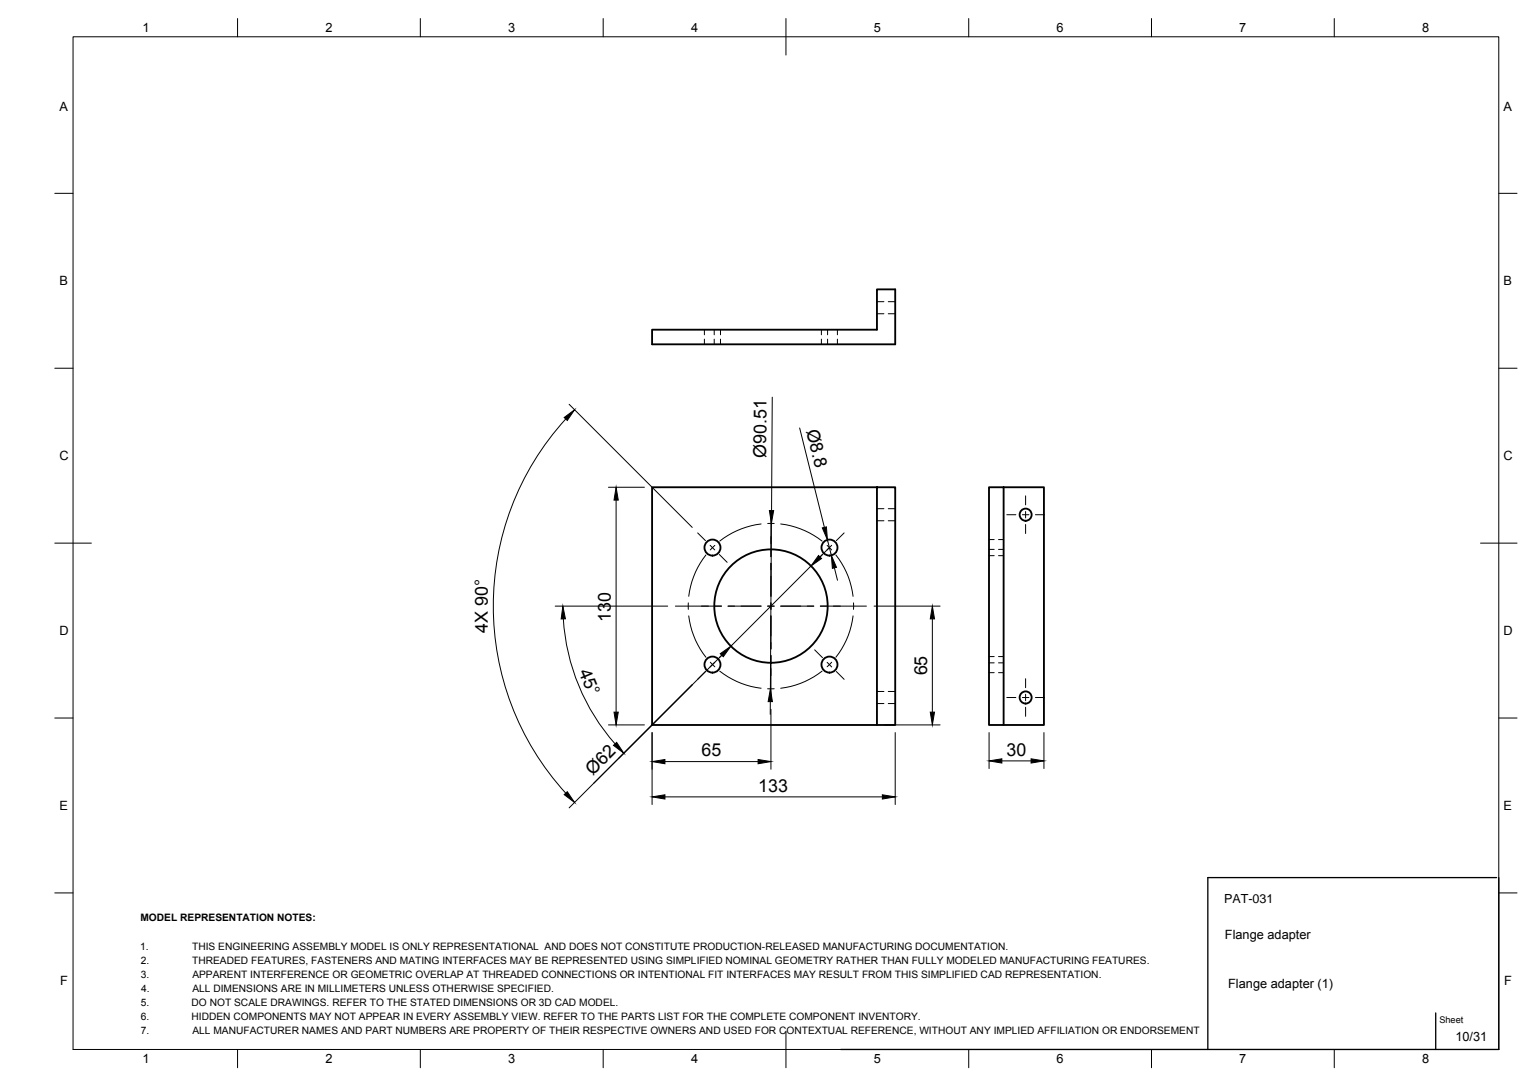
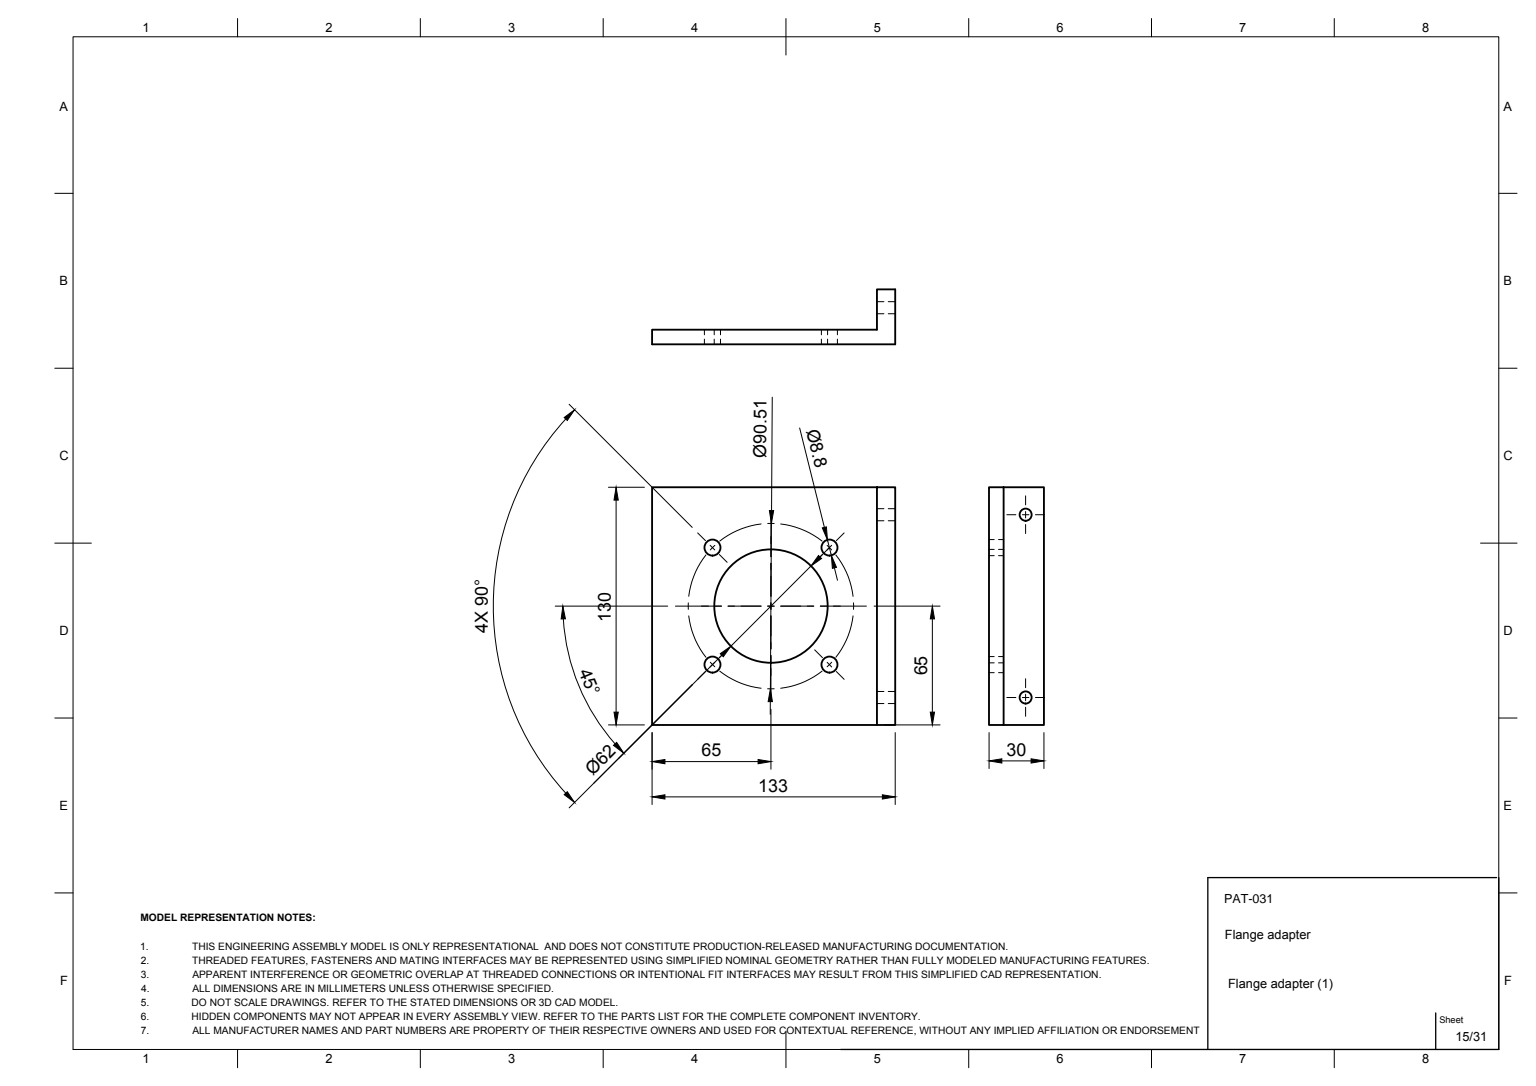
ISO-10303-21;
HEADER;
/* Generated by software containing ST-Developer
 * from STEP Tools, Inc. (www.steptools.com) 
 */

FILE_DESCRIPTION(
/* description */ ('Double-row support with tensioned shaft'),
/* implementation_level */ '2;1');

FILE_NAME(
/* name */ 'Flange adapter.step',
/* time_stamp */ '2026-10-27T10:50:35-07:00',
/* author */ (''),
/* organization */ (''),
/* preprocessor_version */ 'ST-DEVELOPER v20.2',
/* originating_system */ 'Autodesk Translation Framework v15.17.0.0',
/* authorisation */ '');

FILE_SCHEMA (('AUTOMOTIVE_DESIGN { 1 0 10303 214 3 1 1 }'));
ENDSEC;

DATA;
#10=MECHANICAL_DESIGN_GEOMETRIC_PRESENTATION_REPRESENTATION('',(#484),#11559);
#420=SHAPE_REPRESENTATION_RELATIONSHIP('SRR','None',#11728,#452);
#452=ADVANCED_BREP_SHAPE_REPRESENTATION('',(#517),#11530);
#484=STYLED_ITEM('',(#11953),#517);
#517=MANIFOLD_SOLID_BREP('Body1',#6329);
#566=FACE_BOUND('',#1335,.T.);
#567=FACE_BOUND('',#1336,.T.);
#568=FACE_BOUND('',#1339,.T.);
#569=FACE_BOUND('',#1340,.T.);
#570=FACE_BOUND('',#1341,.T.);
#571=FACE_BOUND('',#1342,.T.);
#572=FACE_BOUND('',#1343,.T.);
#573=FACE_BOUND('',#1347,.T.);
#574=FACE_BOUND('',#1348,.T.);
#575=FACE_BOUND('',#1349,.T.);
#576=FACE_BOUND('',#1350,.T.);
#577=FACE_BOUND('',#1351,.T.);
#578=FACE_BOUND('',#1354,.T.);
#579=FACE_BOUND('',#1355,.T.);
#709=PLANE('',#6808);
#710=PLANE('',#6809);
#711=PLANE('',#6810);
#712=PLANE('',#6811);
#713=PLANE('',#6812);
#714=PLANE('',#6813);
#715=PLANE('',#6814);
#716=PLANE('',#6815);
#959=FACE_OUTER_BOUND('',#1327,.T.);
#960=FACE_OUTER_BOUND('',#1328,.T.);
#961=FACE_OUTER_BOUND('',#1329,.T.);
#962=FACE_OUTER_BOUND('',#1330,.T.);
#963=FACE_OUTER_BOUND('',#1331,.T.);
#964=FACE_OUTER_BOUND('',#1332,.T.);
#965=FACE_OUTER_BOUND('',#1333,.T.);
#966=FACE_OUTER_BOUND('',#1334,.T.);
#967=FACE_OUTER_BOUND('',#1337,.T.);
#968=FACE_OUTER_BOUND('',#1338,.T.);
#969=FACE_OUTER_BOUND('',#1344,.T.);
#970=FACE_OUTER_BOUND('',#1345,.T.);
#971=FACE_OUTER_BOUND('',#1346,.T.);
#972=FACE_OUTER_BOUND('',#1352,.T.);
#973=FACE_OUTER_BOUND('',#1353,.T.);
#1327=EDGE_LOOP('',(#4522,#4523,#4524,#4525));
#1328=EDGE_LOOP('',(#4526,#4527,#4528,#4529));
#1329=EDGE_LOOP('',(#4530,#4531,#4532,#4533));
#1330=EDGE_LOOP('',(#4534,#4535,#4536,#4537));
#1331=EDGE_LOOP('',(#4538,#4539,#4540,#4541));
#1332=EDGE_LOOP('',(#4542,#4543,#4544,#4545));
#1333=EDGE_LOOP('',(#4546,#4547,#4548,#4549));
#1334=EDGE_LOOP('',(#4550,#4551,#4552,#4553));
#1335=EDGE_LOOP('',(#4554));
#1336=EDGE_LOOP('',(#4555));
#1337=EDGE_LOOP('',(#4556,#4557,#4558,#4559));
#1338=EDGE_LOOP('',(#4560,#4561,#4562,#4563));
#1339=EDGE_LOOP('',(#4564));
#1340=EDGE_LOOP('',(#4565));
#1341=EDGE_LOOP('',(#4566));
#1342=EDGE_LOOP('',(#4567));
#1343=EDGE_LOOP('',(#4568));
#1344=EDGE_LOOP('',(#4569,#4570,#4571,#4572,#4573,#4574));
#1345=EDGE_LOOP('',(#4575,#4576,#4577,#4578,#4579,#4580));
#1346=EDGE_LOOP('',(#4581,#4582,#4583,#4584));
#1347=EDGE_LOOP('',(#4585));
#1348=EDGE_LOOP('',(#4586));
#1349=EDGE_LOOP('',(#4587));
#1350=EDGE_LOOP('',(#4588));
#1351=EDGE_LOOP('',(#4589));
#1352=EDGE_LOOP('',(#4590,#4591,#4592,#4593));
#1353=EDGE_LOOP('',(#4594,#4595,#4596,#4597));
#1354=EDGE_LOOP('',(#4598));
#1355=EDGE_LOOP('',(#4599));
#1814=LINE('',#9448,#2361);
#1815=LINE('',#9454,#2362);
#1816=LINE('',#9460,#2363);
#1817=LINE('',#9466,#2364);
#1818=LINE('',#9472,#2365);
#1819=LINE('',#9478,#2366);
#1820=LINE('',#9484,#2367);
#1821=LINE('',#9489,#2368);
#1822=LINE('',#9491,#2369);
#1823=LINE('',#9493,#2370);
#1824=LINE('',#9494,#2371);
#1825=LINE('',#9497,#2372);
#1826=LINE('',#9499,#2373);
#1827=LINE('',#9500,#2374);
#1828=LINE('',#9504,#2375);
#1829=LINE('',#9506,#2376);
#1830=LINE('',#9508,#2377);
#1831=LINE('',#9509,#2378);
#1832=LINE('',#9512,#2379);
#1833=LINE('',#9513,#2380);
#1834=LINE('',#9514,#2381);
#1835=LINE('',#9517,#2382);
#1836=LINE('',#9518,#2383);
#1837=LINE('',#9519,#2384);
#1838=LINE('',#9521,#2385);
#2361=VECTOR('',#7595,0.33);
#2362=VECTOR('',#7602,0.33);
#2363=VECTOR('',#7609,0.44);
#2364=VECTOR('',#7616,0.44);
#2365=VECTOR('',#7623,0.44);
#2366=VECTOR('',#7630,0.44);
#2367=VECTOR('',#7637,3.1);
#2368=VECTOR('',#7642,1.);
#2369=VECTOR('',#7643,1.);
#2370=VECTOR('',#7644,1.);
#2371=VECTOR('',#7645,1.);
#2372=VECTOR('',#7648,1.);
#2373=VECTOR('',#7649,1.);
#2374=VECTOR('',#7650,1.);
#2375=VECTOR('',#7653,1.);
#2376=VECTOR('',#7654,1.);
#2377=VECTOR('',#7655,1.);
#2378=VECTOR('',#7656,1.);
#2379=VECTOR('',#7659,1.);
#2380=VECTOR('',#7660,1.);
#2381=VECTOR('',#7661,1.);
#2382=VECTOR('',#7664,1.);
#2383=VECTOR('',#7665,1.);
#2384=VECTOR('',#7666,1.);
#2385=VECTOR('',#7669,1.);
#2860=CIRCLE('',#6788,0.33);
#2861=CIRCLE('',#6789,0.33);
#2862=CIRCLE('',#6791,0.33);
#2863=CIRCLE('',#6792,0.33);
#2864=CIRCLE('',#6794,0.44);
#2865=CIRCLE('',#6795,0.44);
#2866=CIRCLE('',#6797,0.44);
#2867=CIRCLE('',#6798,0.44);
#2868=CIRCLE('',#6800,0.44);
#2869=CIRCLE('',#6801,0.44);
#2870=CIRCLE('',#6803,0.44);
#2871=CIRCLE('',#6804,0.44);
#2872=CIRCLE('',#6806,3.1);
#2873=CIRCLE('',#6807,3.1);
#3091=VERTEX_POINT('',#9445);
#3092=VERTEX_POINT('',#9447);
#3093=VERTEX_POINT('',#9451);
#3094=VERTEX_POINT('',#9453);
#3095=VERTEX_POINT('',#9457);
#3096=VERTEX_POINT('',#9459);
#3097=VERTEX_POINT('',#9463);
#3098=VERTEX_POINT('',#9465);
#3099=VERTEX_POINT('',#9469);
#3100=VERTEX_POINT('',#9471);
#3101=VERTEX_POINT('',#9475);
#3102=VERTEX_POINT('',#9477);
#3103=VERTEX_POINT('',#9481);
#3104=VERTEX_POINT('',#9483);
#3105=VERTEX_POINT('',#9487);
#3106=VERTEX_POINT('',#9488);
#3107=VERTEX_POINT('',#9490);
#3108=VERTEX_POINT('',#9492);
#3109=VERTEX_POINT('',#9496);
#3110=VERTEX_POINT('',#9498);
#3111=VERTEX_POINT('',#9502);
#3112=VERTEX_POINT('',#9503);
#3113=VERTEX_POINT('',#9505);
#3114=VERTEX_POINT('',#9507);
#3115=VERTEX_POINT('',#9511);
#3116=VERTEX_POINT('',#9516);
#3646=EDGE_CURVE('',#3091,#3091,#2860,.T.);
#3647=EDGE_CURVE('',#3091,#3092,#1814,.T.);
#3648=EDGE_CURVE('',#3092,#3092,#2861,.T.);
#3649=EDGE_CURVE('',#3093,#3093,#2862,.T.);
#3650=EDGE_CURVE('',#3093,#3094,#1815,.T.);
#3651=EDGE_CURVE('',#3094,#3094,#2863,.T.);
#3652=EDGE_CURVE('',#3095,#3095,#2864,.T.);
#3653=EDGE_CURVE('',#3095,#3096,#1816,.T.);
#3654=EDGE_CURVE('',#3096,#3096,#2865,.T.);
#3655=EDGE_CURVE('',#3097,#3097,#2866,.T.);
#3656=EDGE_CURVE('',#3097,#3098,#1817,.T.);
#3657=EDGE_CURVE('',#3098,#3098,#2867,.T.);
#3658=EDGE_CURVE('',#3099,#3099,#2868,.T.);
#3659=EDGE_CURVE('',#3099,#3100,#1818,.T.);
#3660=EDGE_CURVE('',#3100,#3100,#2869,.T.);
#3661=EDGE_CURVE('',#3101,#3101,#2870,.T.);
#3662=EDGE_CURVE('',#3101,#3102,#1819,.T.);
#3663=EDGE_CURVE('',#3102,#3102,#2871,.T.);
#3664=EDGE_CURVE('',#3103,#3103,#2872,.T.);
#3665=EDGE_CURVE('',#3103,#3104,#1820,.T.);
#3666=EDGE_CURVE('',#3104,#3104,#2873,.T.);
#3667=EDGE_CURVE('',#3105,#3106,#1821,.T.);
#3668=EDGE_CURVE('',#3107,#3105,#1822,.T.);
#3669=EDGE_CURVE('',#3108,#3107,#1823,.T.);
#3670=EDGE_CURVE('',#3108,#3106,#1824,.T.);
#3671=EDGE_CURVE('',#3107,#3109,#1825,.T.);
#3672=EDGE_CURVE('',#3109,#3110,#1826,.T.);
#3673=EDGE_CURVE('',#3110,#3108,#1827,.T.);
#3674=EDGE_CURVE('',#3111,#3112,#1828,.T.);
#3675=EDGE_CURVE('',#3113,#3112,#1829,.T.);
#3676=EDGE_CURVE('',#3114,#3113,#1830,.T.);
#3677=EDGE_CURVE('',#3114,#3111,#1831,.T.);
#3678=EDGE_CURVE('',#3105,#3115,#1832,.T.);
#3679=EDGE_CURVE('',#3112,#3115,#1833,.T.);
#3680=EDGE_CURVE('',#3111,#3109,#1834,.T.);
#3681=EDGE_CURVE('',#3116,#3113,#1835,.T.);
#3682=EDGE_CURVE('',#3106,#3116,#1836,.T.);
#3683=EDGE_CURVE('',#3110,#3114,#1837,.T.);
#3684=EDGE_CURVE('',#3115,#3116,#1838,.T.);
#4522=ORIENTED_EDGE('',*,*,#3646,.F.);
#4523=ORIENTED_EDGE('',*,*,#3647,.T.);
#4524=ORIENTED_EDGE('',*,*,#3648,.F.);
#4525=ORIENTED_EDGE('',*,*,#3647,.F.);
#4526=ORIENTED_EDGE('',*,*,#3649,.F.);
#4527=ORIENTED_EDGE('',*,*,#3650,.T.);
#4528=ORIENTED_EDGE('',*,*,#3651,.F.);
#4529=ORIENTED_EDGE('',*,*,#3650,.F.);
#4530=ORIENTED_EDGE('',*,*,#3652,.F.);
#4531=ORIENTED_EDGE('',*,*,#3653,.T.);
#4532=ORIENTED_EDGE('',*,*,#3654,.F.);
#4533=ORIENTED_EDGE('',*,*,#3653,.F.);
#4534=ORIENTED_EDGE('',*,*,#3655,.F.);
#4535=ORIENTED_EDGE('',*,*,#3656,.T.);
#4536=ORIENTED_EDGE('',*,*,#3657,.F.);
#4537=ORIENTED_EDGE('',*,*,#3656,.F.);
#4538=ORIENTED_EDGE('',*,*,#3658,.F.);
#4539=ORIENTED_EDGE('',*,*,#3659,.T.);
#4540=ORIENTED_EDGE('',*,*,#3660,.F.);
#4541=ORIENTED_EDGE('',*,*,#3659,.F.);
#4542=ORIENTED_EDGE('',*,*,#3661,.F.);
#4543=ORIENTED_EDGE('',*,*,#3662,.T.);
#4544=ORIENTED_EDGE('',*,*,#3663,.F.);
#4545=ORIENTED_EDGE('',*,*,#3662,.F.);
#4546=ORIENTED_EDGE('',*,*,#3664,.F.);
#4547=ORIENTED_EDGE('',*,*,#3665,.T.);
#4548=ORIENTED_EDGE('',*,*,#3666,.F.);
#4549=ORIENTED_EDGE('',*,*,#3665,.F.);
#4550=ORIENTED_EDGE('',*,*,#3667,.F.);
#4551=ORIENTED_EDGE('',*,*,#3668,.F.);
#4552=ORIENTED_EDGE('',*,*,#3669,.F.);
#4553=ORIENTED_EDGE('',*,*,#3670,.T.);
#4554=ORIENTED_EDGE('',*,*,#3648,.T.);
#4555=ORIENTED_EDGE('',*,*,#3651,.T.);
#4556=ORIENTED_EDGE('',*,*,#3669,.T.);
#4557=ORIENTED_EDGE('',*,*,#3671,.T.);
#4558=ORIENTED_EDGE('',*,*,#3672,.T.);
#4559=ORIENTED_EDGE('',*,*,#3673,.T.);
#4560=ORIENTED_EDGE('',*,*,#3674,.T.);
#4561=ORIENTED_EDGE('',*,*,#3675,.F.);
#4562=ORIENTED_EDGE('',*,*,#3676,.F.);
#4563=ORIENTED_EDGE('',*,*,#3677,.T.);
#4564=ORIENTED_EDGE('',*,*,#3666,.T.);
#4565=ORIENTED_EDGE('',*,*,#3663,.T.);
#4566=ORIENTED_EDGE('',*,*,#3660,.T.);
#4567=ORIENTED_EDGE('',*,*,#3657,.T.);
#4568=ORIENTED_EDGE('',*,*,#3654,.T.);
#4569=ORIENTED_EDGE('',*,*,#3678,.T.);
#4570=ORIENTED_EDGE('',*,*,#3679,.F.);
#4571=ORIENTED_EDGE('',*,*,#3674,.F.);
#4572=ORIENTED_EDGE('',*,*,#3680,.T.);
#4573=ORIENTED_EDGE('',*,*,#3671,.F.);
#4574=ORIENTED_EDGE('',*,*,#3668,.T.);
#4575=ORIENTED_EDGE('',*,*,#3676,.T.);
#4576=ORIENTED_EDGE('',*,*,#3681,.F.);
#4577=ORIENTED_EDGE('',*,*,#3682,.F.);
#4578=ORIENTED_EDGE('',*,*,#3670,.F.);
#4579=ORIENTED_EDGE('',*,*,#3673,.F.);
#4580=ORIENTED_EDGE('',*,*,#3683,.T.);
#4581=ORIENTED_EDGE('',*,*,#3667,.T.);
#4582=ORIENTED_EDGE('',*,*,#3682,.T.);
#4583=ORIENTED_EDGE('',*,*,#3684,.F.);
#4584=ORIENTED_EDGE('',*,*,#3678,.F.);
#4585=ORIENTED_EDGE('',*,*,#3664,.T.);
#4586=ORIENTED_EDGE('',*,*,#3661,.T.);
#4587=ORIENTED_EDGE('',*,*,#3658,.T.);
#4588=ORIENTED_EDGE('',*,*,#3655,.T.);
#4589=ORIENTED_EDGE('',*,*,#3652,.T.);
#4590=ORIENTED_EDGE('',*,*,#3679,.T.);
#4591=ORIENTED_EDGE('',*,*,#3684,.T.);
#4592=ORIENTED_EDGE('',*,*,#3681,.T.);
#4593=ORIENTED_EDGE('',*,*,#3675,.T.);
#4594=ORIENTED_EDGE('',*,*,#3680,.F.);
#4595=ORIENTED_EDGE('',*,*,#3677,.F.);
#4596=ORIENTED_EDGE('',*,*,#3683,.F.);
#4597=ORIENTED_EDGE('',*,*,#3672,.F.);
#4598=ORIENTED_EDGE('',*,*,#3646,.T.);
#4599=ORIENTED_EDGE('',*,*,#3649,.T.);
#5902=CYLINDRICAL_SURFACE('',#6787,0.33);
#5903=CYLINDRICAL_SURFACE('',#6790,0.33);
#5904=CYLINDRICAL_SURFACE('',#6793,0.44);
#5905=CYLINDRICAL_SURFACE('',#6796,0.44);
#5906=CYLINDRICAL_SURFACE('',#6799,0.44);
#5907=CYLINDRICAL_SURFACE('',#6802,0.44);
#5908=CYLINDRICAL_SURFACE('',#6805,3.1);
#6022=ADVANCED_FACE('',(#959),#5902,.F.);
#6023=ADVANCED_FACE('',(#960),#5903,.F.);
#6024=ADVANCED_FACE('',(#961),#5904,.F.);
#6025=ADVANCED_FACE('',(#962),#5905,.F.);
#6026=ADVANCED_FACE('',(#963),#5906,.F.);
#6027=ADVANCED_FACE('',(#964),#5907,.F.);
#6028=ADVANCED_FACE('',(#965),#5908,.F.);
#6029=ADVANCED_FACE('',(#966,#566,#567),#709,.T.);
#6030=ADVANCED_FACE('',(#967),#710,.F.);
#6031=ADVANCED_FACE('',(#968,#568,#569,#570,#571,#572),#711,.T.);
#6032=ADVANCED_FACE('',(#969),#712,.T.);
#6033=ADVANCED_FACE('',(#970),#713,.T.);
#6034=ADVANCED_FACE('',(#971,#573,#574,#575,#576,#577),#714,.T.);
#6035=ADVANCED_FACE('',(#972),#715,.T.);
#6036=ADVANCED_FACE('',(#973,#578,#579),#716,.F.);
#6329=CLOSED_SHELL('',(#6022,#6023,#6024,#6025,#6026,#6027,#6028,#6029,
#6030,#6031,#6032,#6033,#6034,#6035,#6036));
#6786=AXIS2_PLACEMENT_3D('',#9443,#7589,#7590);
#6787=AXIS2_PLACEMENT_3D('',#9444,#7591,#7592);
#6788=AXIS2_PLACEMENT_3D('',#9446,#7593,#7594);
#6789=AXIS2_PLACEMENT_3D('',#9449,#7596,#7597);
#6790=AXIS2_PLACEMENT_3D('',#9450,#7598,#7599);
#6791=AXIS2_PLACEMENT_3D('',#9452,#7600,#7601);
#6792=AXIS2_PLACEMENT_3D('',#9455,#7603,#7604);
#6793=AXIS2_PLACEMENT_3D('',#9456,#7605,#7606);
#6794=AXIS2_PLACEMENT_3D('',#9458,#7607,#7608);
#6795=AXIS2_PLACEMENT_3D('',#9461,#7610,#7611);
#6796=AXIS2_PLACEMENT_3D('',#9462,#7612,#7613);
#6797=AXIS2_PLACEMENT_3D('',#9464,#7614,#7615);
#6798=AXIS2_PLACEMENT_3D('',#9467,#7617,#7618);
#6799=AXIS2_PLACEMENT_3D('',#9468,#7619,#7620);
#6800=AXIS2_PLACEMENT_3D('',#9470,#7621,#7622);
#6801=AXIS2_PLACEMENT_3D('',#9473,#7624,#7625);
#6802=AXIS2_PLACEMENT_3D('',#9474,#7626,#7627);
#6803=AXIS2_PLACEMENT_3D('',#9476,#7628,#7629);
#6804=AXIS2_PLACEMENT_3D('',#9479,#7631,#7632);
#6805=AXIS2_PLACEMENT_3D('',#9480,#7633,#7634);
#6806=AXIS2_PLACEMENT_3D('',#9482,#7635,#7636);
#6807=AXIS2_PLACEMENT_3D('',#9485,#7638,#7639);
#6808=AXIS2_PLACEMENT_3D('',#9486,#7640,#7641);
#6809=AXIS2_PLACEMENT_3D('',#9495,#7646,#7647);
#6810=AXIS2_PLACEMENT_3D('',#9501,#7651,#7652);
#6811=AXIS2_PLACEMENT_3D('',#9510,#7657,#7658);
#6812=AXIS2_PLACEMENT_3D('',#9515,#7662,#7663);
#6813=AXIS2_PLACEMENT_3D('',#9520,#7667,#7668);
#6814=AXIS2_PLACEMENT_3D('',#9522,#7670,#7671);
#6815=AXIS2_PLACEMENT_3D('',#9523,#7672,#7673);
#7589=DIRECTION('axis',(0.,0.,1.));
#7590=DIRECTION('refdir',(1.,0.,0.));
#7591=DIRECTION('center_axis',(0.,0.,1.));
#7592=DIRECTION('ref_axis',(1.,0.,0.));
#7593=DIRECTION('center_axis',(0.,0.,1.));
#7594=DIRECTION('ref_axis',(1.,0.,0.));
#7595=DIRECTION('',(0.,0.,1.));
#7596=DIRECTION('center_axis',(0.,0.,-1.));
#7597=DIRECTION('ref_axis',(1.,0.,0.));
#7598=DIRECTION('center_axis',(0.,0.,1.));
#7599=DIRECTION('ref_axis',(1.,0.,0.));
#7600=DIRECTION('center_axis',(0.,0.,1.));
#7601=DIRECTION('ref_axis',(1.,0.,0.));
#7602=DIRECTION('',(0.,0.,1.));
#7603=DIRECTION('center_axis',(0.,0.,-1.));
#7604=DIRECTION('ref_axis',(1.,0.,0.));
#7605=DIRECTION('center_axis',(0.,1.,0.));
#7606=DIRECTION('ref_axis',(1.,0.,0.));
#7607=DIRECTION('center_axis',(0.,1.,0.));
#7608=DIRECTION('ref_axis',(1.,0.,0.));
#7609=DIRECTION('',(0.,1.,0.));
#7610=DIRECTION('center_axis',(0.,-1.,0.));
#7611=DIRECTION('ref_axis',(1.,0.,0.));
#7612=DIRECTION('center_axis',(0.,1.,0.));
#7613=DIRECTION('ref_axis',(1.,0.,0.));
#7614=DIRECTION('center_axis',(0.,1.,0.));
#7615=DIRECTION('ref_axis',(1.,0.,0.));
#7616=DIRECTION('',(0.,1.,0.));
#7617=DIRECTION('center_axis',(0.,-1.,0.));
#7618=DIRECTION('ref_axis',(1.,0.,0.));
#7619=DIRECTION('center_axis',(0.,1.,0.));
#7620=DIRECTION('ref_axis',(1.,0.,0.));
#7621=DIRECTION('center_axis',(0.,1.,0.));
#7622=DIRECTION('ref_axis',(1.,0.,0.));
#7623=DIRECTION('',(0.,1.,0.));
#7624=DIRECTION('center_axis',(0.,-1.,0.));
#7625=DIRECTION('ref_axis',(1.,0.,0.));
#7626=DIRECTION('center_axis',(0.,1.,0.));
#7627=DIRECTION('ref_axis',(1.,0.,0.));
#7628=DIRECTION('center_axis',(0.,1.,0.));
#7629=DIRECTION('ref_axis',(1.,0.,0.));
#7630=DIRECTION('',(0.,1.,0.));
#7631=DIRECTION('center_axis',(0.,-1.,0.));
#7632=DIRECTION('ref_axis',(1.,0.,0.));
#7633=DIRECTION('center_axis',(0.,1.,0.));
#7634=DIRECTION('ref_axis',(1.,0.,0.));
#7635=DIRECTION('center_axis',(0.,1.,0.));
#7636=DIRECTION('ref_axis',(1.,0.,0.));
#7637=DIRECTION('',(0.,1.,0.));
#7638=DIRECTION('center_axis',(0.,-1.,0.));
#7639=DIRECTION('ref_axis',(1.,0.,0.));
#7640=DIRECTION('center_axis',(0.,0.,1.));
#7641=DIRECTION('ref_axis',(1.,0.,0.));
#7642=DIRECTION('',(1.,0.,0.));
#7643=DIRECTION('',(0.,1.,0.));
#7644=DIRECTION('',(-1.,0.,0.));
#7645=DIRECTION('',(0.,1.,0.));
#7646=DIRECTION('center_axis',(0.,1.,0.));
#7647=DIRECTION('ref_axis',(1.,0.,0.));
#7648=DIRECTION('',(0.,0.,-1.));
#7649=DIRECTION('',(1.,0.,0.));
#7650=DIRECTION('',(0.,0.,1.));
#7651=DIRECTION('center_axis',(0.,1.,0.));
#7652=DIRECTION('ref_axis',(-1.,0.,0.));
#7653=DIRECTION('',(0.,0.,1.));
#7654=DIRECTION('',(-1.,0.,0.));
#7655=DIRECTION('',(0.,0.,1.));
#7656=DIRECTION('',(-1.,0.,0.));
#7657=DIRECTION('center_axis',(-1.,0.,0.));
#7658=DIRECTION('ref_axis',(0.,-1.,0.));
#7659=DIRECTION('',(0.,0.,1.));
#7660=DIRECTION('',(0.,-1.,0.));
#7661=DIRECTION('',(0.,-1.,0.));
#7662=DIRECTION('center_axis',(1.,0.,0.));
#7663=DIRECTION('ref_axis',(0.,1.,0.));
#7664=DIRECTION('',(0.,1.,0.));
#7665=DIRECTION('',(0.,0.,1.));
#7666=DIRECTION('',(0.,1.,0.));
#7667=DIRECTION('center_axis',(0.,-1.,0.));
#7668=DIRECTION('ref_axis',(1.,0.,0.));
#7669=DIRECTION('',(1.,0.,0.));
#7670=DIRECTION('center_axis',(0.,0.,1.));
#7671=DIRECTION('ref_axis',(1.,0.,0.));
#7672=DIRECTION('center_axis',(0.,0.,1.));
#7673=DIRECTION('ref_axis',(1.,0.,0.));
#9443=CARTESIAN_POINT('',(0.,0.,0.));
#9444=CARTESIAN_POINT('Origin',(-5.,-2.5,3.1));
#9445=CARTESIAN_POINT('',(-5.33,-2.5,3.2));
#9446=CARTESIAN_POINT('Origin',(-5.,-2.5,3.2));
#9447=CARTESIAN_POINT('',(-5.33,-2.5,4.2));
#9448=CARTESIAN_POINT('',(-5.33,-2.5,3.1));
#9449=CARTESIAN_POINT('Origin',(-5.,-2.5,4.2));
#9450=CARTESIAN_POINT('Origin',(5.,-2.5,3.1));
#9451=CARTESIAN_POINT('',(4.67,-2.5,3.2));
#9452=CARTESIAN_POINT('Origin',(5.,-2.5,3.2));
#9453=CARTESIAN_POINT('',(4.67,-2.5,4.2));
#9454=CARTESIAN_POINT('',(4.67,-2.5,3.1));
#9455=CARTESIAN_POINT('Origin',(5.,-2.5,4.2));
#9456=CARTESIAN_POINT('Origin',(3.2,-1.4,6.8));
#9457=CARTESIAN_POINT('',(2.76,-1.3,6.8));
#9458=CARTESIAN_POINT('Origin',(3.2,-1.3,6.8));
#9459=CARTESIAN_POINT('',(2.76,-0.5,6.8));
#9460=CARTESIAN_POINT('',(2.76,-1.4,6.8));
#9461=CARTESIAN_POINT('Origin',(3.2,-0.5,6.8));
#9462=CARTESIAN_POINT('Origin',(-3.2,-1.4,13.2));
#9463=CARTESIAN_POINT('',(-3.64,-1.3,13.2));
#9464=CARTESIAN_POINT('Origin',(-3.2,-1.3,13.2));
#9465=CARTESIAN_POINT('',(-3.64,-0.5,13.2));
#9466=CARTESIAN_POINT('',(-3.64,-1.4,13.2));
#9467=CARTESIAN_POINT('Origin',(-3.2,-0.5,13.2));
#9468=CARTESIAN_POINT('Origin',(-3.2,-1.4,6.8));
#9469=CARTESIAN_POINT('',(-3.64,-1.3,6.8));
#9470=CARTESIAN_POINT('Origin',(-3.2,-1.3,6.8));
#9471=CARTESIAN_POINT('',(-3.64,-0.5,6.8));
#9472=CARTESIAN_POINT('',(-3.64,-1.4,6.8));
#9473=CARTESIAN_POINT('Origin',(-3.2,-0.5,6.8));
#9474=CARTESIAN_POINT('Origin',(3.2,-1.4,13.2));
#9475=CARTESIAN_POINT('',(2.76,-1.3,13.2));
#9476=CARTESIAN_POINT('Origin',(3.2,-1.3,13.2));
#9477=CARTESIAN_POINT('',(2.76,-0.5,13.2));
#9478=CARTESIAN_POINT('',(2.76,-1.4,13.2));
#9479=CARTESIAN_POINT('Origin',(3.2,-0.5,13.2));
#9480=CARTESIAN_POINT('Origin',(0.,-1.4,10.));
#9481=CARTESIAN_POINT('',(-3.1,-1.3,10.));
#9482=CARTESIAN_POINT('Origin',(0.,-1.3,10.));
#9483=CARTESIAN_POINT('',(-3.1,-0.5,10.));
#9484=CARTESIAN_POINT('',(-3.1,-1.4,10.));
#9485=CARTESIAN_POINT('Origin',(0.,-0.5,10.));
#9486=CARTESIAN_POINT('Origin',(-6.5,-3.5,4.2));
#9487=CARTESIAN_POINT('',(-6.5,-1.3,4.2));
#9488=CARTESIAN_POINT('',(6.5,-1.3,4.2));
#9489=CARTESIAN_POINT('',(-6.5,-1.3,4.2));
#9490=CARTESIAN_POINT('',(-6.5,-3.5,4.2));
#9491=CARTESIAN_POINT('',(-6.5,-3.5,4.2));
#9492=CARTESIAN_POINT('',(6.5,-3.5,4.2));
#9493=CARTESIAN_POINT('',(6.5,-3.5,4.2));
#9494=CARTESIAN_POINT('',(6.5,-3.5,4.2));
#9495=CARTESIAN_POINT('Origin',(0.,-3.5,3.7));
#9496=CARTESIAN_POINT('',(-6.5,-3.5,3.2));
#9497=CARTESIAN_POINT('',(-6.5,-3.5,4.2));
#9498=CARTESIAN_POINT('',(6.5,-3.5,3.2));
#9499=CARTESIAN_POINT('',(-6.5,-3.5,3.2));
#9500=CARTESIAN_POINT('',(6.5,-3.5,3.2));
#9501=CARTESIAN_POINT('Origin',(6.5,-0.5,3.2));
#9502=CARTESIAN_POINT('',(-6.5,-0.5,3.2));
#9503=CARTESIAN_POINT('',(-6.5,-0.5,16.5));
#9504=CARTESIAN_POINT('',(-6.5,-0.5,3.2));
#9505=CARTESIAN_POINT('',(6.5,-0.5,16.5));
#9506=CARTESIAN_POINT('',(6.5,-0.5,16.5));
#9507=CARTESIAN_POINT('',(6.5,-0.5,3.2));
#9508=CARTESIAN_POINT('',(6.5,-0.5,3.2));
#9509=CARTESIAN_POINT('',(6.5,-0.5,3.2));
#9510=CARTESIAN_POINT('Origin',(-6.5,-0.5,3.2));
#9511=CARTESIAN_POINT('',(-6.5,-1.3,16.5));
#9512=CARTESIAN_POINT('',(-6.5,-1.3,3.2));
#9513=CARTESIAN_POINT('',(-6.5,-0.5,16.5));
#9514=CARTESIAN_POINT('',(-6.5,-0.5,3.2));
#9515=CARTESIAN_POINT('Origin',(6.5,-1.3,3.2));
#9516=CARTESIAN_POINT('',(6.5,-1.3,16.5));
#9517=CARTESIAN_POINT('',(6.5,-1.3,16.5));
#9518=CARTESIAN_POINT('',(6.5,-1.3,3.2));
#9519=CARTESIAN_POINT('',(6.5,-3.5,3.2));
#9520=CARTESIAN_POINT('Origin',(-6.5,-1.3,3.2));
#9521=CARTESIAN_POINT('',(-6.5,-1.3,16.5));
#9522=CARTESIAN_POINT('Origin',(0.,-0.9,16.5));
#9523=CARTESIAN_POINT('Origin',(0.,-0.9,3.2));
#11493=UNCERTAINTY_MEASURE_WITH_UNIT(LENGTH_MEASURE(0.001),#11560,
'DISTANCE_ACCURACY_VALUE',
'Maximum model space distance between geometric entities at asserted c
onnectivities');
#11522=UNCERTAINTY_MEASURE_WITH_UNIT(LENGTH_MEASURE(0.001),#11560,
'DISTANCE_ACCURACY_VALUE',
'Maximum model space distance between geometric entities at asserted c
onnectivities');
#11530=(
GEOMETRIC_REPRESENTATION_CONTEXT(3)
GLOBAL_UNCERTAINTY_ASSIGNED_CONTEXT((#11493))
GLOBAL_UNIT_ASSIGNED_CONTEXT((#11560,#11562,#11563))
REPRESENTATION_CONTEXT('','3D')
);
#11559=(
GEOMETRIC_REPRESENTATION_CONTEXT(3)
GLOBAL_UNCERTAINTY_ASSIGNED_CONTEXT((#11522))
GLOBAL_UNIT_ASSIGNED_CONTEXT((#11560,#11562,#11563))
REPRESENTATION_CONTEXT('','3D')
);
#11560=(
LENGTH_UNIT()
NAMED_UNIT(*)
SI_UNIT(.CENTI.,.METRE.)
);
#11562=(
NAMED_UNIT(*)
PLANE_ANGLE_UNIT()
SI_UNIT($,.RADIAN.)
);
#11563=(
NAMED_UNIT(*)
SI_UNIT($,.STERADIAN.)
SOLID_ANGLE_UNIT()
);
#11571=SHAPE_DEFINITION_REPRESENTATION(#11607,#11728);
#11607=PRODUCT_DEFINITION_SHAPE('',$,#11765);
#11728=SHAPE_REPRESENTATION('',(#6786),#11530);
#11757=PRODUCT_DEFINITION_CONTEXT('part definition',#11867,'design');
#11765=PRODUCT_DEFINITION('Flange adapter','Flange adapter',#11801,#11757);
#11801=PRODUCT_DEFINITION_FORMATION('',$,#11876);
#11867=APPLICATION_CONTEXT(
'Core Data for Automotive Mechanical Design Process');
#11868=PRODUCT_CONTEXT('part definition',#11867,'mechanical');
#11876=PRODUCT('Flange adapter','Flange adapter','Flange adapter',(#11868));
#11947=COLOUR_RGB('Light Blue',0.38,0.62,0.78);
#11948=FILL_AREA_STYLE_COLOUR('',#11947);
#11949=FILL_AREA_STYLE('',(#11948));
#11950=SURFACE_STYLE_FILL_AREA(#11949);
#11951=SURFACE_SIDE_STYLE('',(#11950));
#11952=SURFACE_STYLE_USAGE(.BOTH.,#11951);
#11953=PRESENTATION_STYLE_ASSIGNMENT((#11952));
ENDSEC;
END-ISO-10303-21;
